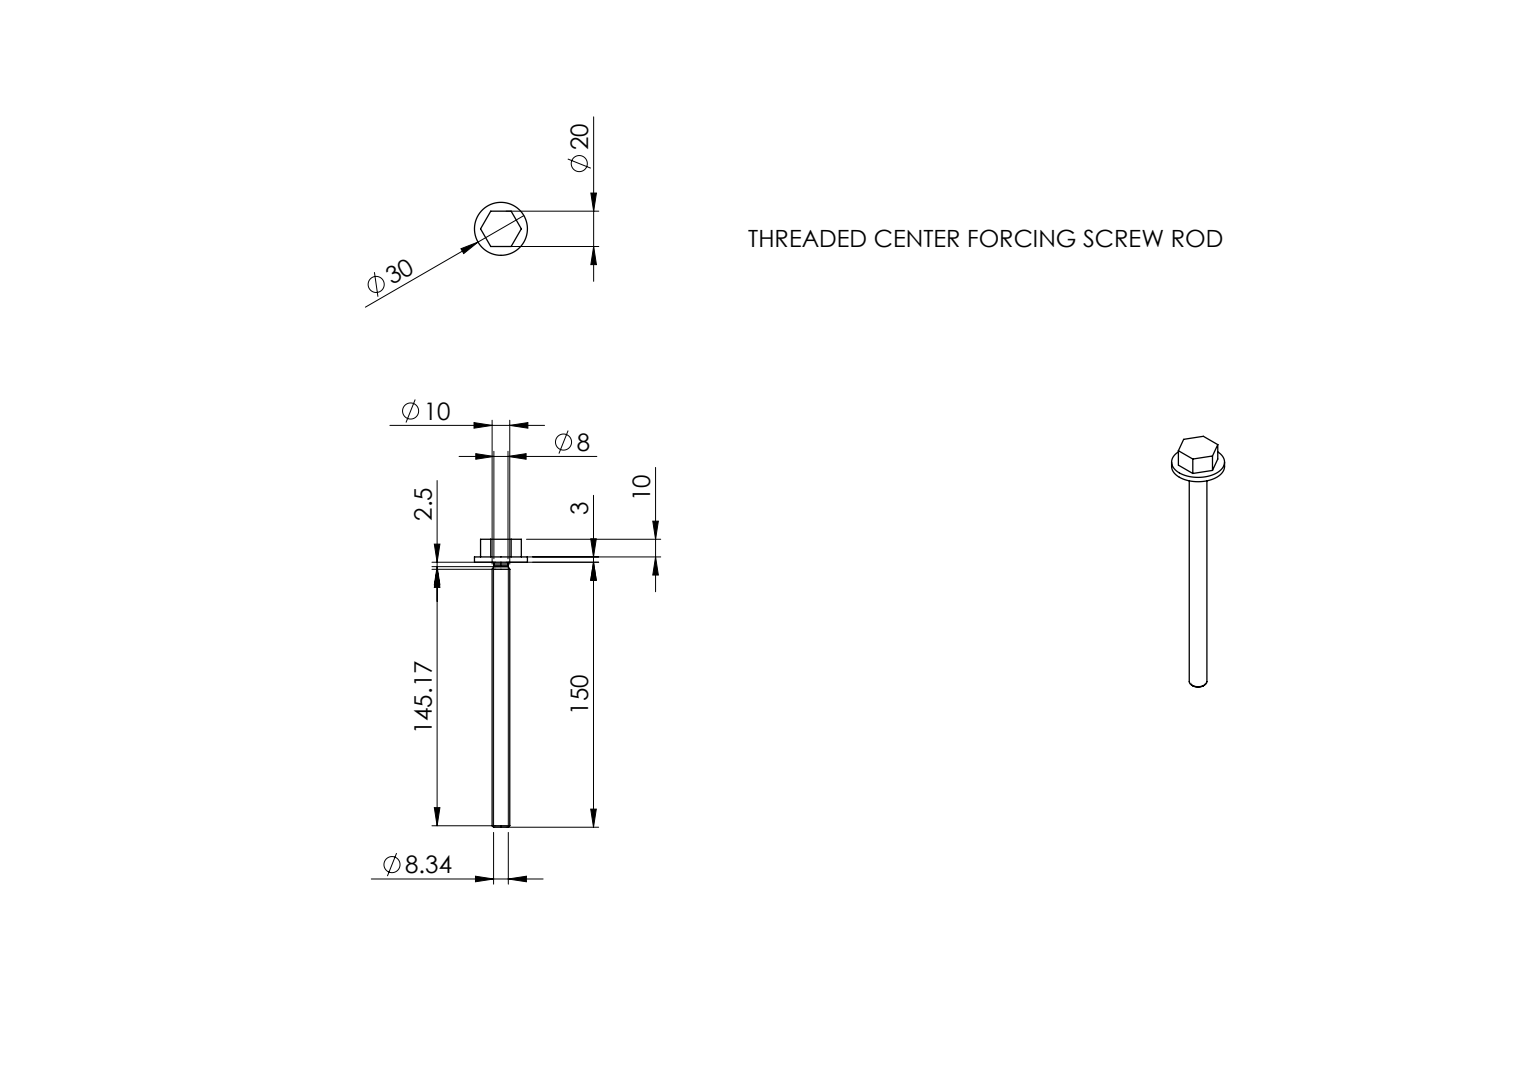
ISO-10303-21;
HEADER;
FILE_DESCRIPTION (('STEP AP214'),
    '1' );
FILE_NAME ('Threaded Center Forcing Screw Rod.step',
    '2026-10-22T13:24:12',
    ( '' ),
    ( '' ),
    'SwSTEP 2.0',
    'SolidWorks 2026',
    '' );
FILE_SCHEMA (( 'AUTOMOTIVE_DESIGN' ));
ENDSEC;

DATA;
#2=CARTESIAN_POINT ( 'NONE',  ( 0.000000000000000000, -150.0000000000000000, 0.000000000000000000 ) ) ;
#4=EDGE_CURVE ( 'NONE', #2839, #391, #2268, .T. ) ;
#5=LINE ( 'NONE', #437, #2768 ) ;
#11=AXIS2_PLACEMENT_3D ( 'NONE', #480, #2053, #1136 ) ;
#12=CARTESIAN_POINT ( 'NONE',  ( 5.510910596163087583E-16, -0.9999999999999997780, -3.999999999999999112 ) ) ;
#14=DIRECTION ( 'NONE',  ( -1.000000000000000000, 0.000000000000000000, 1.502314598737159524E-16 ) ) ;
#17=DIRECTION ( 'NONE',  ( -1.000000000000000000, 0.000000000000000000, 3.004629197474320528E-16 ) ) ;
#18=DIRECTION ( 'NONE',  ( -0.000000000000000000, -1.000000000000000000, -0.000000000000000000 ) ) ;
#24=DIRECTION ( 'NONE',  ( 0.000000000000000000, 0.7071067811865452413, 0.7071067811865497932 ) ) ;
#27=CARTESIAN_POINT ( 'NONE',  ( -5.773502691896258199, 13.00000000000000178, -9.999999999999998224 ) ) ;
#28=EDGE_CURVE ( 'NONE', #2653, #1371, #1839, .T. ) ;
#36=EDGE_CURVE ( 'NONE', #1503, #53, #2280, .T. ) ;
#39=DIRECTION ( 'NONE',  ( -1.000000000000000000, 0.000000000000000000, 0.000000000000000000 ) ) ;
#45=FACE_OUTER_BOUND ( 'NONE', #672, .T. ) ;
#46=AXIS2_PLACEMENT_3D ( 'NONE', #1452, #789, #2135 ) ;
#51=AXIS2_PLACEMENT_3D ( 'NONE', #933, #1833, #2774 ) ;
#53=VERTEX_POINT ( 'NONE', #12 ) ;
#56=CARTESIAN_POINT ( 'NONE',  ( 0.000000000000000000, -1.000000000000000000, 0.000000000000000000 ) ) ;
#71=CIRCLE ( 'NONE', #1705, 4.999999999999998224 ) ;
#74=ORIENTED_EDGE ( 'NONE', *, *, #1121, .T. ) ;
#81=VERTEX_POINT ( 'NONE', #86 ) ;
#85=ORIENTED_EDGE ( 'NONE', *, *, #1055, .F. ) ;
#86=CARTESIAN_POINT ( 'NONE',  ( 0.000000000000000000, -149.1719999999999970, 5.000000000000000000 ) ) ;
#88=ORIENTED_EDGE ( 'NONE', *, *, #2477, .T. ) ;
#90=DIRECTION ( 'NONE',  ( 0.8660254037844383745, 0.000000000000000000, -0.5000000000000004441 ) ) ;
#95=PLANE ( 'NONE',  #2598 ) ;
#96=EDGE_LOOP ( 'NONE', ( #402, #361, #2058, #215 ) ) ;
#107=VECTOR ( 'NONE', #1157, 1000.000000000000000 ) ;
#122=LINE ( 'NONE', #1519, #2601 ) ;
#126=DIRECTION ( 'NONE',  ( -0.8660254037844390407, 0.000000000000000000, -0.4999999999999993339 ) ) ;
#136=DIRECTION ( 'NONE',  ( 0.000000000000000000, 0.000000000000000000, 1.000000000000000000 ) ) ;
#137=DIRECTION ( 'NONE',  ( 0.000000000000000000, 0.000000000000000000, 1.000000000000000000 ) ) ;
#141=AXIS2_PLACEMENT_3D ( 'NONE', #801, #2592, #136 ) ;
#142=EDGE_CURVE ( 'NONE', #1729, #1249, #2519, .T. ) ;
#145=TOROIDAL_SURFACE ( 'NONE', #1548, 4.999999999999998224, 0.9999999999999995559 ) ;
#149=ORIENTED_EDGE ( 'NONE', *, *, #1965, .T. ) ;
#153=CYLINDRICAL_SURFACE ( 'NONE', #1179, 3.999999999999998224 ) ;
#164=EDGE_CURVE ( 'NONE', #1727, #2749, #1701, .T. ) ;
#172=CYLINDRICAL_SURFACE ( 'NONE', #2274, 3.999999999999998224 ) ;
#184=ORIENTED_EDGE ( 'NONE', *, *, #1754, .T. ) ;
#207=FILL_AREA_STYLE_COLOUR ( '', #2269 ) ;
#215=ORIENTED_EDGE ( 'NONE', *, *, #2027, .T. ) ;
#217=DIRECTION ( 'NONE',  ( 0.000000000000000000, -0.000000000000000000, 1.000000000000000000 ) ) ;
#222=EDGE_LOOP ( 'NONE', ( #1224, #1858, #149, #2137 ) ) ;
#226=ORIENTED_EDGE ( 'NONE', *, *, #1897, .F. ) ;
#231=CARTESIAN_POINT ( 'NONE',  ( 0.000000000000000000, 0.000000000000000000, 0.000000000000000000 ) ) ;
#236=VECTOR ( 'NONE', #2191, 1000.000000000000000 ) ;
#240=CIRCLE ( 'NONE', #693, 5.000000000000000000 ) ;
#250=ORIENTED_EDGE ( 'NONE', *, *, #1132, .T. ) ;
#253=CARTESIAN_POINT ( 'NONE',  ( -11.54700538379251107, 13.00000000000000178, 3.469741003519073858E-15 ) ) ;
#260=LINE ( 'NONE', #2310, #780 ) ;
#262=CARTESIAN_POINT ( 'NONE',  ( 0.000000000000000000, 0.000000000000000000, -15.00000000000000178 ) ) ;
#265=CARTESIAN_POINT ( 'NONE',  ( -5.773502691896248429, 3.000000000000000000, 10.00000000000000178 ) ) ;
#268=CARTESIAN_POINT ( 'NONE',  ( 5.773502691896260863, 13.00000000000000178, 9.999999999999998224 ) ) ;
#280=ADVANCED_FACE ( 'NONE', ( #1721 ), #153, .T. ) ;
#286=DIRECTION ( 'NONE',  ( 0.000000000000000000, 0.000000000000000000, 1.000000000000000000 ) ) ;
#290=EDGE_LOOP ( 'NONE', ( #622, #1114 ) ) ;
#291=AXIS2_PLACEMENT_3D ( 'NONE', #2036, #2498, #1316 ) ;
#298=DIRECTION ( 'NONE',  ( 0.4999999999999998890, 0.000000000000000000, 0.8660254037844385966 ) ) ;
#301=DIRECTION ( 'NONE',  ( -0.000000000000000000, 1.000000000000000000, -0.000000000000000000 ) ) ;
#306=CARTESIAN_POINT ( 'NONE',  ( 0.000000000000000000, 0.000000000000000000, 0.000000000000000000 ) ) ;
#309=ADVANCED_FACE ( 'NONE', ( #2460 ), #828, .T. ) ;
#310=UNCERTAINTY_MEASURE_WITH_UNIT (LENGTH_MEASURE( 1.000000000000000082E-05 ), #2495, 'distance_accuracy_value', 'NONE');
#312=PLANE ( 'NONE',  #1216 ) ;
#329=CARTESIAN_POINT ( 'NONE',  ( 5.773502691896260863, 13.00000000000000178, 9.999999999999998224 ) ) ;
#330=EDGE_LOOP ( 'NONE', ( #811, #74, #1656, #2066 ) ) ;
#337=LINE ( 'NONE', #1932, #2374 ) ;
#338=DIRECTION ( 'NONE',  ( -0.000000000000000000, 1.000000000000000000, -0.000000000000000000 ) ) ;
#342=PRODUCT_DEFINITION ( 'UNKNOWN', '', #694, #2622 ) ;
#350=CARTESIAN_POINT ( 'NONE',  ( 0.000000000000000000, -2.500000000000000444, 0.000000000000000000 ) ) ;
#351=EDGE_LOOP ( 'NONE', ( #2396, #1986, #2575, #2754 ) ) ;
#358=EDGE_LOOP ( 'NONE', ( #85, #2337, #684, #88 ) ) ;
#360=FACE_OUTER_BOUND ( 'NONE', #424, .T. ) ;
#361=ORIENTED_EDGE ( 'NONE', *, *, #1809, .F. ) ;
#365=ORIENTED_EDGE ( 'NONE', *, *, #2096, .T. ) ;
#375=EDGE_CURVE ( 'NONE', #957, #1371, #1659, .T. ) ;
#382=ORIENTED_EDGE ( 'NONE', *, *, #2069, .F. ) ;
#391=VERTEX_POINT ( 'NONE', #1838 ) ;
#402=ORIENTED_EDGE ( 'NONE', *, *, #1276, .T. ) ;
#404=LINE ( 'NONE', #1296, #697 ) ;
#405=ADVANCED_FACE ( 'NONE', ( #1352 ), #696, .T. ) ;
#406=DIRECTION ( 'NONE',  ( 0.000000000000000000, 0.000000000000000000, 1.000000000000000000 ) ) ;
#414=( NAMED_UNIT ( * ) SI_UNIT ( $, .STERADIAN. ) SOLID_ANGLE_UNIT ( ) );
#420=LINE ( 'NONE', #253, #2911 ) ;
#421=VECTOR ( 'NONE', #2760, 1000.000000000000227 ) ;
#423=CIRCLE ( 'NONE', #2414, 4.171999999999999709 ) ;
#424=EDGE_LOOP ( 'NONE', ( #674, #785, #2678, #603 ) ) ;
#428=CARTESIAN_POINT ( 'NONE',  ( 0.000000000000000000, -2.500000000000000444, 0.000000000000000000 ) ) ;
#431=( NAMED_UNIT ( * ) SI_UNIT ( $, .STERADIAN. ) SOLID_ANGLE_UNIT ( ) );
#437=CARTESIAN_POINT ( 'NONE',  ( -5.773502691896248429, 13.00000000000000178, 10.00000000000000178 ) ) ;
#447=CARTESIAN_POINT ( 'NONE',  ( 0.000000000000000000, -2.500000000000000444, 4.133974596215572284 ) ) ;
#453=DIRECTION ( 'NONE',  ( -0.000000000000000000, 1.000000000000000000, -0.000000000000000000 ) ) ;
#457=ADVANCED_FACE ( 'NONE', ( #955 ), #1807, .T. ) ;
#459=ORIENTED_EDGE ( 'NONE', *, *, #2639, .T. ) ;
#479=EDGE_CURVE ( 'NONE', #1049, #81, #1573, .T. ) ;
#480=CARTESIAN_POINT ( 'NONE',  ( 5.773502691896257311, 13.00000000000000178, -10.00000000000000000 ) ) ;
#494=LINE ( 'NONE', #2776, #516 ) ;
#499=ORIENTED_EDGE ( 'NONE', *, *, #1348, .T. ) ;
#505=DIRECTION ( 'NONE',  ( -0.000000000000000000, 1.000000000000000000, -0.000000000000000000 ) ) ;
#507=VECTOR ( 'NONE', #1679, 1000.000000000000000 ) ;
#516=VECTOR ( 'NONE', #2323, 1000.000000000000000 ) ;
#517=DIRECTION ( 'NONE',  ( -0.000000000000000000, 1.000000000000000000, -0.000000000000000000 ) ) ;
#524=DIRECTION ( 'NONE',  ( 0.4999999999999993339, 0.000000000000000000, -0.8660254037844390407 ) ) ;
#530=ORIENTED_EDGE ( 'NONE', *, *, #2477, .F. ) ;
#537=DIRECTION ( 'NONE',  ( 0.000000000000000000, -0.000000000000000000, 1.000000000000000000 ) ) ;
#541=CARTESIAN_POINT ( 'NONE',  ( 6.123233995736766282E-16, -149.1719999999999970, -5.000000000000000000 ) ) ;
#543=DIRECTION ( 'NONE',  ( 0.000000000000000000, 1.000000000000000000, 0.000000000000000000 ) ) ;
#547=FACE_OUTER_BOUND ( 'NONE', #614, .T. ) ;
#548=FACE_OUTER_BOUND ( 'NONE', #2786, .T. ) ;
#551=ORIENTED_EDGE ( 'NONE', *, *, #1102, .F. ) ;
#555=CARTESIAN_POINT ( 'NONE',  ( 0.000000000000000000, 0.000000000000000000, 3.999999999999998224 ) ) ;
#577=APPLICATION_CONTEXT ( 'automotive_design' ) ;
#579=EDGE_CURVE ( 'NONE', #2653, #2728, #1992, .T. ) ;
#603=ORIENTED_EDGE ( 'NONE', *, *, #1774, .T. ) ;
#612=CARTESIAN_POINT ( 'NONE',  ( 0.000000000000000000, -2.500000000000000444, 0.000000000000000000 ) ) ;
#613=AXIS2_PLACEMENT_3D ( 'NONE', #2778, #2490, #1152 ) ;
#614=EDGE_LOOP ( 'NONE', ( #226, #2248, #1244, #2777 ) ) ;
#622=ORIENTED_EDGE ( 'NONE', *, *, #1348, .F. ) ;
#631=EDGE_LOOP ( 'NONE', ( #499, #763, #2072, #2015 ) ) ;
#637=ORIENTED_EDGE ( 'NONE', *, *, #2069, .T. ) ;
#639=DIRECTION ( 'NONE',  ( 0.000000000000000000, 1.000000000000000000, 0.000000000000000000 ) ) ;
#641=VECTOR ( 'NONE', #1326, 1000.000000000000000 ) ;
#643=ORIENTED_EDGE ( 'NONE', *, *, #2783, .T. ) ;
#656=ORIENTED_EDGE ( 'NONE', *, *, #1809, .T. ) ;
#670=LINE ( 'NONE', #1066, #641 ) ;
#672=EDGE_LOOP ( 'NONE', ( #2930, #1394, #2851, #2536 ) ) ;
#673=CARTESIAN_POINT ( 'NONE',  ( 0.000000000000000000, 3.000000000000000000, -15.00000000000000178 ) ) ;
#674=ORIENTED_EDGE ( 'NONE', *, *, #2651, .F. ) ;
#675=CARTESIAN_POINT ( 'NONE',  ( 5.773502691896260863, 3.000000000000000000, 9.999999999999998224 ) ) ;
#684=ORIENTED_EDGE ( 'NONE', *, *, #1451, .T. ) ;
#686=DIRECTION ( 'NONE',  ( -0.000000000000000000, 1.000000000000000000, -0.000000000000000000 ) ) ;
#693=AXIS2_PLACEMENT_3D ( 'NONE', #1251, #2832, #2860 ) ;
#694=PRODUCT_DEFINITION_FORMATION_WITH_SPECIFIED_SOURCE ( 'ANY', '', #2336, .NOT_KNOWN. ) ;
#696=PLANE ( 'NONE',  #708 ) ;
#697=VECTOR ( 'NONE', #2211, 1000.000000000000000 ) ;
#700=DIRECTION ( 'NONE',  ( 0.000000000000000000, -0.8660254037844267172, -0.5000000000000207612 ) ) ;
#701=AXIS2_PLACEMENT_3D ( 'NONE', #1280, #1697, #2617 ) ;
#705=VERTEX_POINT ( 'NONE', #1582 ) ;
#708=AXIS2_PLACEMENT_3D ( 'NONE', #1588, #2746, #1605 ) ;
#709=DIRECTION ( 'NONE',  ( 1.224646799147352468E-16, 0.000000000000000000, -1.000000000000000000 ) ) ;
#710=PLANE ( 'NONE',  #2891 ) ;
#711=PLANE ( 'NONE',  #2371 ) ;
#714=ORIENTED_EDGE ( 'NONE', *, *, #1505, .F. ) ;
#720=ORIENTED_EDGE ( 'NONE', *, *, #2117, .F. ) ;
#723=DIRECTION ( 'NONE',  ( 0.000000000000000000, 0.000000000000000000, 1.000000000000000000 ) ) ;
#734=CARTESIAN_POINT ( 'NONE',  ( 0.000000000000000000, -1.999999999999980016, 0.000000000000000000 ) ) ;
#735=CARTESIAN_POINT ( 'NONE',  ( 0.000000000000000000, 0.000000000000000000, 0.000000000000000000 ) ) ;
#737=VERTEX_POINT ( 'NONE', #1314 ) ;
#745=DIRECTION ( 'NONE',  ( -0.000000000000000000, -1.000000000000000000, -0.000000000000000000 ) ) ;
#754=CLOSED_SHELL ( 'NONE', ( #2881, #457, #2145, #2721, #1585, #2277, #1625, #2040, #2699, #1248, #2372, #1234, #1321, #2735, #2694, #1354, #2112, #1825, #280, #1540, #2775, #309, #1255, #405 ) ) ;
#756=EDGE_LOOP ( 'NONE', ( #1133, #2308, #2005, #864 ) ) ;
#759=ORIENTED_EDGE ( 'NONE', *, *, #1412, .F. ) ;
#763=ORIENTED_EDGE ( 'NONE', *, *, #2164, .T. ) ;
#766=VERTEX_POINT ( 'NONE', #675 ) ;
#771=DIRECTION ( 'NONE',  ( -0.4999999999999996114, 0.000000000000000000, 0.8660254037844388186 ) ) ;
#774=FACE_OUTER_BOUND ( 'NONE', #1288, .T. ) ;
#775=DIRECTION ( 'NONE',  ( 0.000000000000000000, 0.000000000000000000, 1.000000000000000000 ) ) ;
#776=VERTEX_POINT ( 'NONE', #2729 ) ;
#780=VECTOR ( 'NONE', #700, 1000.000000000000114 ) ;
#781=DIRECTION ( 'NONE',  ( -0.4999999999999996114, 0.000000000000000000, 0.8660254037844388186 ) ) ;
#784=VECTOR ( 'NONE', #2823, 1000.000000000000114 ) ;
#785=ORIENTED_EDGE ( 'NONE', *, *, #375, .F. ) ;
#789=DIRECTION ( 'NONE',  ( -0.000000000000000000, 1.000000000000000000, -0.000000000000000000 ) ) ;
#793=DIRECTION ( 'NONE',  ( -0.000000000000000000, 1.000000000000000000, -0.000000000000000000 ) ) ;
#801=CARTESIAN_POINT ( 'NONE',  ( 0.000000000000000000, 0.000000000000000000, 0.000000000000000000 ) ) ;
#806=CYLINDRICAL_SURFACE ( 'NONE', #1212, 15.00000000000000178 ) ;
#809=DIRECTION ( 'NONE',  ( -0.000000000000000000, 1.000000000000000000, -0.000000000000000000 ) ) ;
#811=ORIENTED_EDGE ( 'NONE', *, *, #1012, .F. ) ;
#828=CYLINDRICAL_SURFACE ( 'NONE', #2090, 5.000000000000000000 ) ;
#829=VECTOR ( 'NONE', #2691, 1000.000000000000227 ) ;
#830=FACE_OUTER_BOUND ( 'NONE', #1229, .T. ) ;
#835=DIRECTION ( 'NONE',  ( 0.000000000000000000, 0.000000000000000000, -1.000000000000000000 ) ) ;
#847=DIRECTION ( 'NONE',  ( -0.000000000000000000, 1.000000000000000000, -0.000000000000000000 ) ) ;
#864=ORIENTED_EDGE ( 'NONE', *, *, #1102, .T. ) ;
#882=AXIS2_PLACEMENT_3D ( 'NONE', #2250, #639, #217 ) ;
#885=CIRCLE ( 'NONE', #2702, 15.00000000000000178 ) ;
#894=AXIS2_PLACEMENT_3D ( 'NONE', #2, #2007, #2052 ) ;
#902=AXIS2_PLACEMENT_3D ( 'NONE', #2158, #1001, #137 ) ;
#907=LINE ( 'NONE', #1297, #2385 ) ;
#911=ORIENTED_EDGE ( 'NONE', *, *, #36, .T. ) ;
#915=VERTEX_POINT ( 'NONE', #265 ) ;
#919=DIRECTION ( 'NONE',  ( -0.8660254037844387076, 0.000000000000000000, 0.4999999999999999445 ) ) ;
#933=CARTESIAN_POINT ( 'NONE',  ( 0.000000000000000000, -1.000000000000000000, 4.999999999999998224 ) ) ;
#934=CIRCLE ( 'NONE', #141, 4.999999999999998224 ) ;
#939=CIRCLE ( 'NONE', #291, 1.000000000000000000 ) ;
#943=DIRECTION ( 'NONE',  ( -0.000000000000000000, 1.000000000000000000, -0.000000000000000000 ) ) ;
#949=CARTESIAN_POINT ( 'NONE',  ( 0.000000000000000000, -0.9999999999999997780, 3.999999999999999112 ) ) ;
#950=PLANE ( 'NONE',  #2507 ) ;
#953=VECTOR ( 'NONE', #2121, 1000.000000000000000 ) ;
#955=FACE_OUTER_BOUND ( 'NONE', #1436, .T. ) ;
#957=VERTEX_POINT ( 'NONE', #961 ) ;
#958=DIRECTION ( 'NONE',  ( -0.000000000000000000, -1.000000000000000000, -0.000000000000000000 ) ) ;
#961=CARTESIAN_POINT ( 'NONE',  ( 5.062658757011871940E-16, -2.500000000000000444, -4.133974596215572284 ) ) ;
#963=CARTESIAN_POINT ( 'NONE',  ( -11.54700538379251107, 13.00000000000000178, 3.469741003519073858E-15 ) ) ;
#976=DIRECTION ( 'NONE',  ( -0.5000000000000004441, 0.000000000000000000, -0.8660254037844383745 ) ) ;
#978=CIRCLE ( 'NONE', #46, 3.999999999999999112 ) ;
#983=DIRECTION ( 'NONE',  ( -0.4999999999999993339, 0.000000000000000000, 0.8660254037844390407 ) ) ;
#990=LINE ( 'NONE', #2821, #953 ) ;
#992=CARTESIAN_POINT ( 'NONE',  ( 0.000000000000000000, -1.999999999999980016, 3.999999999999998224 ) ) ;
#1001=DIRECTION ( 'NONE',  ( -0.000000000000000000, 1.000000000000000000, -0.000000000000000000 ) ) ;
#1002=FACE_OUTER_BOUND ( 'NONE', #358, .T. ) ;
#1005=CARTESIAN_POINT ( 'NONE',  ( 0.000000000000000000, -149.1719999999999970, 0.000000000000000000 ) ) ;
#1006=ORIENTED_EDGE ( 'NONE', *, *, #1311, .F. ) ;
#1012=EDGE_CURVE ( 'NONE', #2433, #2749, #990, .T. ) ;
#1040=CARTESIAN_POINT ( 'NONE',  ( 0.000000000000000000, 0.000000000000000000, 0.000000000000000000 ) ) ;
#1045=CARTESIAN_POINT ( 'NONE',  ( 11.54700538379251107, 13.00000000000000178, -6.939586148520149327E-15 ) ) ;
#1049=VERTEX_POINT ( 'NONE', #1350 ) ;
#1055=EDGE_CURVE ( 'NONE', #1249, #1871, #1541, .T. ) ;
#1060=EDGE_LOOP ( 'NONE', ( #2209, #1680, #1329, #656 ) ) ;
#1065=EDGE_CURVE ( 'NONE', #1905, #776, #420, .T. ) ;
#1066=CARTESIAN_POINT ( 'NONE',  ( 6.123233995736766282E-16, -149.1719999999999970, -5.000000000000000000 ) ) ;
#1069=CONICAL_SURFACE ( 'NONE', #1688, 5.000000000000000000, 0.7853981633974514986 ) ;
#1070=DIRECTION ( 'NONE',  ( -0.000000000000000000, -1.000000000000000000, -0.000000000000000000 ) ) ;
#1078=CARTESIAN_POINT ( 'NONE',  ( 0.000000000000000000, -149.1719999999999970, 0.000000000000000000 ) ) ;
#1088=CIRCLE ( 'NONE', #2620, 5.000000000000000000 ) ;
#1090=SURFACE_STYLE_USAGE ( .BOTH. , #2467 ) ;
#1094=DIRECTION ( 'NONE',  ( -0.000000000000000000, 1.000000000000000000, -0.000000000000000000 ) ) ;
#1102=EDGE_CURVE ( 'NONE', #2075, #766, #907, .T. ) ;
#1108=PLANE ( 'NONE',  #1552 ) ;
#1109=DIRECTION ( 'NONE',  ( -0.000000000000000000, -1.000000000000000000, -0.000000000000000000 ) ) ;
#1113=DIRECTION ( 'NONE',  ( -0.000000000000000000, 1.000000000000000000, -0.000000000000000000 ) ) ;
#1114=ORIENTED_EDGE ( 'NONE', *, *, #1749, .F. ) ;
#1115=CONICAL_SURFACE ( 'NONE', #1495, 4.133974596215571395, 0.5235987755983229075 ) ;
#1116=DIRECTION ( 'NONE',  ( -0.000000000000000000, 1.000000000000000000, -0.000000000000000000 ) ) ;
#1118=VECTOR ( 'NONE', #781, 1000.000000000000114 ) ;
#1121=EDGE_CURVE ( 'NONE', #2433, #81, #1088, .T. ) ;
#1124=CIRCLE ( 'NONE', #2810, 5.000000000000000000 ) ;
#1126=CARTESIAN_POINT ( 'NONE',  ( 0.000000000000000000, -149.1719999999999970, 5.000000000000000000 ) ) ;
#1129=LINE ( 'NONE', #2046, #2025 ) ;
#1132=EDGE_CURVE ( 'NONE', #705, #1494, #71, .T. ) ;
#1133=ORIENTED_EDGE ( 'NONE', *, *, #2872, .T. ) ;
#1136=DIRECTION ( 'NONE',  ( 1.000000000000000000, 0.000000000000000000, -1.502314598737159524E-16 ) ) ;
#1137=PLANE ( 'NONE',  #11 ) ;
#1138=EDGE_CURVE ( 'NONE', #776, #915, #5, .T. ) ;
#1152=DIRECTION ( 'NONE',  ( 0.000000000000000000, 0.000000000000000000, 1.000000000000000000 ) ) ;
#1156=CARTESIAN_POINT ( 'NONE',  ( 0.000000000000000000, -1.999999999999980016, 4.999999999999998224 ) ) ;
#1157=DIRECTION ( 'NONE',  ( -0.000000000000000000, -1.000000000000000000, -0.000000000000000000 ) ) ;
#1160=VECTOR ( 'NONE', #745, 1000.000000000000000 ) ;
#1170=( GEOMETRIC_REPRESENTATION_CONTEXT ( 3 ) GLOBAL_UNCERTAINTY_ASSIGNED_CONTEXT ( ( #1831 ) ) GLOBAL_UNIT_ASSIGNED_CONTEXT ( ( #1477, #2599, #2403 ) ) REPRESENTATION_CONTEXT ( 'NONE', 'WORKASPACE' ) );
#1173=TOROIDAL_SURFACE ( 'NONE', #2177, 4.999999999999998224, 0.9999999999999995559 ) ;
#1176=ADVANCED_BREP_SHAPE_REPRESENTATION ( '', ( #1577, #2652 ), #2217 ) ;
#1177=ORIENTED_EDGE ( 'NONE', *, *, #2449, .F. ) ;
#1179=AXIS2_PLACEMENT_3D ( 'NONE', #1498, #847, #2190 ) ;
#1182=DIRECTION ( 'NONE',  ( 0.000000000000000000, 1.000000000000000000, 0.000000000000000000 ) ) ;
#1192=DIRECTION ( 'NONE',  ( 0.000000000000000000, 0.000000000000000000, 1.000000000000000000 ) ) ;
#1197=DIRECTION ( 'NONE',  ( 1.000000000000000000, 0.000000000000000000, 1.224646799147353207E-16 ) ) ;
#1199=LINE ( 'NONE', #268, #1313 ) ;
#1207=ORIENTED_EDGE ( 'NONE', *, *, #1276, .F. ) ;
#1209=UNCERTAINTY_MEASURE_WITH_UNIT (LENGTH_MEASURE( 1.000000000000000082E-05 ), #1985, 'distance_accuracy_value', 'NONE');
#1212=AXIS2_PLACEMENT_3D ( 'NONE', #2643, #1709, #2630 ) ;
#1216=AXIS2_PLACEMENT_3D ( 'NONE', #963, #90, #976 ) ;
#1222=MECHANICAL_DESIGN_GEOMETRIC_PRESENTATION_REPRESENTATION('',(#2563),#1170);
#1224=ORIENTED_EDGE ( 'NONE', *, *, #2639, .F. ) ;
#1226=AXIS2_PLACEMENT_3D ( 'NONE', #1911, #543, #2398 ) ;
#1229=EDGE_LOOP ( 'NONE', ( #720, #2771, #2825, #2871 ) ) ;
#1233=ORIENTED_EDGE ( 'NONE', *, *, #28, .T. ) ;
#1234=ADVANCED_FACE ( 'NONE', ( #2307 ), #2083, .F. ) ;
#1235=VECTOR ( 'NONE', #1109, 1000.000000000000000 ) ;
#1238=DIRECTION ( 'NONE',  ( -0.000000000000000000, 1.000000000000000000, -0.000000000000000000 ) ) ;
#1244=ORIENTED_EDGE ( 'NONE', *, *, #1840, .T. ) ;
#1247=LINE ( 'NONE', #555, #2262 ) ;
#1248=ADVANCED_FACE ( 'NONE', ( #2533, #2743 ), #711, .F. ) ;
#1249=VERTEX_POINT ( 'NONE', #1834 ) ;
#1251=CARTESIAN_POINT ( 'NONE',  ( 0.000000000000000000, -149.1719999999999970, 0.000000000000000000 ) ) ;
#1255=ADVANCED_FACE ( 'NONE', ( #45 ), #1463, .T. ) ;
#1260=STYLED_ITEM ( 'NONE', ( #1770 ), #1176 ) ;
#1261=CARTESIAN_POINT ( 'NONE',  ( 5.773502691896260863, 13.00000000000000178, 9.999999999999998224 ) ) ;
#1265=DIRECTION ( 'NONE',  ( 0.000000000000000000, 0.000000000000000000, 1.000000000000000000 ) ) ;
#1271=CIRCLE ( 'NONE', #1370, 15.00000000000000178 ) ;
#1276=EDGE_CURVE ( 'NONE', #1425, #737, #494, .T. ) ;
#1279=EDGE_LOOP ( 'NONE', ( #530, #2658 ) ) ;
#1280=CARTESIAN_POINT ( 'NONE',  ( 0.000000000000000000, -1.999999999999980016, 0.000000000000000000 ) ) ;
#1281=DIRECTION ( 'NONE',  ( 0.5000000000000004441, 0.000000000000000000, 0.8660254037844383745 ) ) ;
#1286=EDGE_CURVE ( 'NONE', #2075, #2839, #1199, .T. ) ;
#1288=EDGE_LOOP ( 'NONE', ( #759, #2631, #1233, #2088 ) ) ;
#1296=CARTESIAN_POINT ( 'NONE',  ( 0.000000000000000000, 3.000000000000000000, -15.00000000000000178 ) ) ;
#1297=CARTESIAN_POINT ( 'NONE',  ( 5.773502691896260863, 13.00000000000000178, 9.999999999999998224 ) ) ;
#1298=EDGE_LOOP ( 'NONE', ( #2796, #1177 ) ) ;
#1304=FACE_OUTER_BOUND ( 'NONE', #1611, .T. ) ;
#1307=AXIS2_PLACEMENT_3D ( 'NONE', #350, #1726, #835 ) ;
#1309=DIRECTION ( 'NONE',  ( 1.000000000000000000, 0.000000000000000000, 0.000000000000000000 ) ) ;
#1311=EDGE_CURVE ( 'NONE', #391, #1425, #1853, .T. ) ;
#1313=VECTOR ( 'NONE', #524, 1000.000000000000000 ) ;
#1314=CARTESIAN_POINT ( 'NONE',  ( -5.773502691896258199, 3.000000000000000000, -9.999999999999998224 ) ) ;
#1316=DIRECTION ( 'NONE',  ( 1.224646799147352468E-16, 0.000000000000000000, -1.000000000000000000 ) ) ;
#1321=ADVANCED_FACE ( 'NONE', ( #2354 ), #1137, .F. ) ;
#1326=DIRECTION ( 'NONE',  ( 8.659560562354961208E-17, 0.7071067811865452413, -0.7071067811865497932 ) ) ;
#1329=ORIENTED_EDGE ( 'NONE', *, *, #2351, .F. ) ;
#1340=LINE ( 'NONE', #1734, #236 ) ;
#1348=EDGE_CURVE ( 'NONE', #1049, #2555, #2607, .T. ) ;
#1350=CARTESIAN_POINT ( 'NONE',  ( 0.000000000000000000, -150.0000000000000000, 4.171999999999999709 ) ) ;
#1352=FACE_OUTER_BOUND ( 'NONE', #290, .T. ) ;
#1353=SHAPE_DEFINITION_REPRESENTATION ( #1870, #1689 ) ;
#1354=ADVANCED_FACE ( 'NONE', ( #2487 ), #1108, .F. ) ;
#1356=AXIS2_PLACEMENT_3D ( 'NONE', #1821, #453, #286 ) ;
#1357=ORIENTED_EDGE ( 'NONE', *, *, #1012, .T. ) ;
#1359=CARTESIAN_POINT ( 'NONE',  ( 0.000000000000000000, -150.0000000000000000, 0.000000000000000000 ) ) ;
#1361=ORIENTED_EDGE ( 'NONE', *, *, #1897, .T. ) ;
#1362=CIRCLE ( 'NONE', #1460, 3.999999999999998224 ) ;
#1366=CARTESIAN_POINT ( 'NONE',  ( 5.773502691896257311, 3.000000000000000000, -10.00000000000000000 ) ) ;
#1370=AXIS2_PLACEMENT_3D ( 'NONE', #306, #1845, #1192 ) ;
#1371=VERTEX_POINT ( 'NONE', #447 ) ;
#1372=DIRECTION ( 'NONE',  ( -0.000000000000000000, 1.000000000000000000, -0.000000000000000000 ) ) ;
#1392=DIRECTION ( 'NONE',  ( 0.000000000000000000, 0.000000000000000000, 1.000000000000000000 ) ) ;
#1394=ORIENTED_EDGE ( 'NONE', *, *, #1749, .T. ) ;
#1398=LINE ( 'NONE', #1864, #2504 ) ;
#1409=CIRCLE ( 'NONE', #2885, 15.00000000000000178 ) ;
#1412=EDGE_CURVE ( 'NONE', #2728, #957, #939, .T. ) ;
#1422=AXIS2_PLACEMENT_3D ( 'NONE', #2726, #1070, #2483 ) ;
#1425=VERTEX_POINT ( 'NONE', #1366 ) ;
#1426=CARTESIAN_POINT ( 'NONE',  ( -5.773502691896258199, 13.00000000000000178, -9.999999999999998224 ) ) ;
#1436=EDGE_LOOP ( 'NONE', ( #643, #1357, #2693, #2857 ) ) ;
#1437=DIRECTION ( 'NONE',  ( 0.000000000000000000, 0.000000000000000000, 1.000000000000000000 ) ) ;
#1451=EDGE_CURVE ( 'NONE', #1729, #1842, #404, .T. ) ;
#1452=CARTESIAN_POINT ( 'NONE',  ( 0.000000000000000000, -0.9999999999999997780, 0.000000000000000000 ) ) ;
#1455=CARTESIAN_POINT ( 'NONE',  ( 0.000000000000000000, -1.999999999999980016, 0.000000000000000000 ) ) ;
#1457=ORIENTED_EDGE ( 'NONE', *, *, #28, .F. ) ;
#1460=AXIS2_PLACEMENT_3D ( 'NONE', #734, #338, #2063 ) ;
#1463=CONICAL_SURFACE ( 'NONE', #2174, 5.000000000000000000, 0.7853981633974514986 ) ;
#1477=( LENGTH_UNIT ( ) NAMED_UNIT ( * ) SI_UNIT ( .MILLI., .METRE. ) );
#1481=ORIENTED_EDGE ( 'NONE', *, *, #1138, .T. ) ;
#1487=DIRECTION ( 'NONE',  ( 1.000000000000000000, 0.000000000000000000, -3.004629197474320528E-16 ) ) ;
#1494=VERTEX_POINT ( 'NONE', #1644 ) ;
#1495=AXIS2_PLACEMENT_3D ( 'NONE', #612, #2708, #2900 ) ;
#1498=CARTESIAN_POINT ( 'NONE',  ( 0.000000000000000000, 0.000000000000000000, 0.000000000000000000 ) ) ;
#1500=CONICAL_SURFACE ( 'NONE', #1307, 4.133974596215571395, 0.5235987755983229075 ) ;
#1503=VERTEX_POINT ( 'NONE', #949 ) ;
#1505=EDGE_CURVE ( 'NONE', #1494, #53, #2224, .T. ) ;
#1513=DIRECTION ( 'NONE',  ( -0.000000000000000000, 1.000000000000000000, -0.000000000000000000 ) ) ;
#1515=PRODUCT_CONTEXT ( 'NONE', #577, 'mechanical' ) ;
#1519=CARTESIAN_POINT ( 'NONE',  ( 5.773502691896260863, 3.000000000000000000, 9.999999999999998224 ) ) ;
#1540=ADVANCED_FACE ( 'NONE', ( #774 ), #2465, .F. ) ;
#1541=LINE ( 'NONE', #2455, #1235 ) ;
#1545=DIRECTION ( 'NONE',  ( 0.000000000000000000, 0.000000000000000000, 1.000000000000000000 ) ) ;
#1548=AXIS2_PLACEMENT_3D ( 'NONE', #1455, #2367, #723 ) ;
#1552=AXIS2_PLACEMENT_3D ( 'NONE', #2684, #2714, #17 ) ;
#1560=EDGE_CURVE ( 'NONE', #81, #1727, #337, .T. ) ;
#1570=ORIENTED_EDGE ( 'NONE', *, *, #1967, .T. ) ;
#1573=LINE ( 'NONE', #1126, #2856 ) ;
#1577=MANIFOLD_SOLID_BREP ( 'M10 Machine Threads Stud1', #754 ) ;
#1580=( NAMED_UNIT ( * ) PLANE_ANGLE_UNIT ( ) SI_UNIT ( $, .RADIAN. ) );
#1582=CARTESIAN_POINT ( 'NONE',  ( 0.000000000000000000, -2.168404344971008868E-16, 4.999999999999998224 ) ) ;
#1585=ADVANCED_FACE ( 'NONE', ( #2859 ), #172, .T. ) ;
#1588=CARTESIAN_POINT ( 'NONE',  ( 4.171999999999999709, -150.0000000000000000, 0.000000000000000000 ) ) ;
#1590=VECTOR ( 'NONE', #1487, 1000.000000000000000 ) ;
#1593=CARTESIAN_POINT ( 'NONE',  ( -11.54700538379251107, 13.00000000000000178, 3.469741003519073858E-15 ) ) ;
#1601=ORIENTED_EDGE ( 'NONE', *, *, #1965, .F. ) ;
#1604=ORIENTED_EDGE ( 'NONE', *, *, #2732, .F. ) ;
#1605=DIRECTION ( 'NONE',  ( 0.000000000000000000, -0.000000000000000000, -1.000000000000000000 ) ) ;
#1611=EDGE_LOOP ( 'NONE', ( #1682, #1948, #184, #2392, #1977, #637 ) ) ;
#1614=CARTESIAN_POINT ( 'NONE',  ( -5.773502691896258199, 13.00000000000000178, -9.999999999999998224 ) ) ;
#1616=DIRECTION ( 'NONE',  ( 0.000000000000000000, 0.000000000000000000, 1.000000000000000000 ) ) ;
#1624=DIRECTION ( 'NONE',  ( 0.000000000000000000, 0.000000000000000000, 1.000000000000000000 ) ) ;
#1625=ADVANCED_FACE ( 'NONE', ( #547 ), #2366, .T. ) ;
#1633=ORIENTED_EDGE ( 'NONE', *, *, #1065, .F. ) ;
#1641=EDGE_LOOP ( 'NONE', ( #714, #2345, #1793, #911 ) ) ;
#1644=CARTESIAN_POINT ( 'NONE',  ( 6.123233995736764310E-16, -2.168404344971008868E-16, -4.999999999999998224 ) ) ;
#1646=CARTESIAN_POINT ( 'NONE',  ( 11.54700538379251107, 13.00000000000000178, -6.939586148520149327E-15 ) ) ;
#1656=ORIENTED_EDGE ( 'NONE', *, *, #1560, .T. ) ;
#1659=CIRCLE ( 'NONE', #613, 4.133974596215571395 ) ;
#1661=LINE ( 'NONE', #2589, #784 ) ;
#1664=ORIENTED_EDGE ( 'NONE', *, *, #2845, .F. ) ;
#1674=FACE_BOUND ( 'NONE', #2662, .T. ) ;
#1679=DIRECTION ( 'NONE',  ( -0.000000000000000000, -1.000000000000000000, -0.000000000000000000 ) ) ;
#1680=ORIENTED_EDGE ( 'NONE', *, *, #1914, .F. ) ;
#1682=ORIENTED_EDGE ( 'NONE', *, *, #1286, .T. ) ;
#1688=AXIS2_PLACEMENT_3D ( 'NONE', #1005, #1907, #775 ) ;
#1689=SHAPE_REPRESENTATION ( 'Threaded Center Forcing Screw Rod', ( #2652 ), #2217 ) ;
#1697=DIRECTION ( 'NONE',  ( -0.000000000000000000, 1.000000000000000000, -0.000000000000000000 ) ) ;
#1701=CIRCLE ( 'NONE', #902, 5.000000000000000000 ) ;
#1705=AXIS2_PLACEMENT_3D ( 'NONE', #2913, #2500, #406 ) ;
#1709=DIRECTION ( 'NONE',  ( -0.000000000000000000, -1.000000000000000000, -0.000000000000000000 ) ) ;
#1721=FACE_OUTER_BOUND ( 'NONE', #222, .T. ) ;
#1726=DIRECTION ( 'NONE',  ( 0.000000000000000000, -1.000000000000000000, 0.000000000000000000 ) ) ;
#1727=VERTEX_POINT ( 'NONE', #2924 ) ;
#1729=VERTEX_POINT ( 'NONE', #673 ) ;
#1734=CARTESIAN_POINT ( 'NONE',  ( -5.773502691896248429, 3.000000000000000000, 10.00000000000000178 ) ) ;
#1735=AXIS2_PLACEMENT_3D ( 'NONE', #1646, #919, #298 ) ;
#1740=DIRECTION ( 'NONE',  ( 0.000000000000000000, 0.000000000000000000, 1.000000000000000000 ) ) ;
#1745=DIRECTION ( 'NONE',  ( -0.000000000000000000, -1.000000000000000000, -0.000000000000000000 ) ) ;
#1749=EDGE_CURVE ( 'NONE', #2555, #1049, #423, .T. ) ;
#1754=EDGE_CURVE ( 'NONE', #2644, #1806, #2665, .T. ) ;
#1767=CARTESIAN_POINT ( 'NONE',  ( 11.54700538379251107, 13.00000000000000178, -6.939586148520149327E-15 ) ) ;
#1768=ORIENTED_EDGE ( 'NONE', *, *, #2845, .T. ) ;
#1770=PRESENTATION_STYLE_ASSIGNMENT (( #1090 ) ) ;
#1774=EDGE_CURVE ( 'NONE', #2749, #1727, #1124, .T. ) ;
#1793=ORIENTED_EDGE ( 'NONE', *, *, #2732, .T. ) ;
#1798=CARTESIAN_POINT ( 'NONE',  ( 5.773502691896257311, 13.00000000000000178, -10.00000000000000000 ) ) ;
#1806=VERTEX_POINT ( 'NONE', #27 ) ;
#1807=CYLINDRICAL_SURFACE ( 'NONE', #2905, 5.000000000000000000 ) ;
#1809=EDGE_CURVE ( 'NONE', #1806, #737, #2287, .T. ) ;
#1811=DIRECTION ( 'NONE',  ( 0.000000000000000000, 0.000000000000000000, 1.000000000000000000 ) ) ;
#1812=SHAPE_REPRESENTATION_RELATIONSHIP ( 'NONE' , 'NONE' ,  #1689, #1176 ) ;
#1817=CARTESIAN_POINT ( 'NONE',  ( 0.000000000000000000, -149.1719999999999970, 0.000000000000000000 ) ) ;
#1821=CARTESIAN_POINT ( 'NONE',  ( 0.000000000000000000, -1.000000000000000000, 0.000000000000000000 ) ) ;
#1825=ADVANCED_FACE ( 'NONE', ( #2074 ), #1173, .F. ) ;
#1829=CIRCLE ( 'NONE', #51, 1.000000000000000000 ) ;
#1831=UNCERTAINTY_MEASURE_WITH_UNIT (LENGTH_MEASURE( 1.000000000000000082E-05 ), #1477, 'distance_accuracy_value', 'NONE');
#1833=DIRECTION ( 'NONE',  ( -1.000000000000000000, 0.000000000000000000, 0.000000000000000000 ) ) ;
#1834=CARTESIAN_POINT ( 'NONE',  ( 1.836970198721029983E-15, 3.000000000000000000, 15.00000000000000178 ) ) ;
#1838=CARTESIAN_POINT ( 'NONE',  ( 11.54700538379251107, 3.000000000000000000, -6.939586148520149327E-15 ) ) ;
#1839=CIRCLE ( 'NONE', #2329, 1.000000000000000000 ) ;
#1840=EDGE_CURVE ( 'NONE', #1871, #1842, #1271, .T. ) ;
#1842=VERTEX_POINT ( 'NONE', #262 ) ;
#1843=DIRECTION ( 'NONE',  ( 0.000000000000000000, 0.000000000000000000, 1.000000000000000000 ) ) ;
#1845=DIRECTION ( 'NONE',  ( 0.000000000000000000, 1.000000000000000000, 0.000000000000000000 ) ) ;
#1852=CARTESIAN_POINT ( 'NONE',  ( 0.000000000000000000, 3.000000000000000000, 0.000000000000000000 ) ) ;
#1853=LINE ( 'NONE', #2518, #421 ) ;
#1858=ORIENTED_EDGE ( 'NONE', *, *, #2722, .T. ) ;
#1860=CARTESIAN_POINT ( 'NONE',  ( 1.836970198721029983E-15, 0.000000000000000000, 15.00000000000000178 ) ) ;
#1864=CARTESIAN_POINT ( 'NONE',  ( 4.898587196589410857E-16, 0.000000000000000000, -3.999999999999998224 ) ) ;
#1865=DIRECTION ( 'NONE',  ( -0.000000000000000000, 1.000000000000000000, -0.000000000000000000 ) ) ;
#1870=PRODUCT_DEFINITION_SHAPE ( 'NONE', 'NONE',  #342 ) ;
#1871=VERTEX_POINT ( 'NONE', #1860 ) ;
#1873=LINE ( 'NONE', #2803, #1160 ) ;
#1874=TOROIDAL_SURFACE ( 'NONE', #1356, 4.999999999999998224, 0.9999999999999995559 ) ;
#1879=FACE_OUTER_BOUND ( 'NONE', #1898, .T. ) ;
#1892=EDGE_LOOP ( 'NONE', ( #2849, #459, #2162, #1601 ) ) ;
#1897=EDGE_CURVE ( 'NONE', #1249, #1729, #1409, .T. ) ;
#1898=EDGE_LOOP ( 'NONE', ( #1909, #1361 ) ) ;
#1901=CARTESIAN_POINT ( 'NONE',  ( -5.773502691896258199, 13.00000000000000178, -9.999999999999998224 ) ) ;
#1905=VERTEX_POINT ( 'NONE', #1593 ) ;
#1907=DIRECTION ( 'NONE',  ( -0.000000000000000000, 1.000000000000000000, -0.000000000000000000 ) ) ;
#1909=ORIENTED_EDGE ( 'NONE', *, *, #142, .T. ) ;
#1911=CARTESIAN_POINT ( 'NONE',  ( 0.000000000000000000, 3.000000000000000000, 0.000000000000000000 ) ) ;
#1912=LINE ( 'NONE', #2837, #1590 ) ;
#1914=EDGE_CURVE ( 'NONE', #1905, #2512, #1873, .T. ) ;
#1918=CIRCLE ( 'NONE', #2168, 4.133974596215571395 ) ;
#1928=EDGE_CURVE ( 'NONE', #737, #2512, #1129, .T. ) ;
#1930=CARTESIAN_POINT ( 'NONE',  ( 5.773502691896257311, 13.00000000000000178, -10.00000000000000000 ) ) ;
#1932=CARTESIAN_POINT ( 'NONE',  ( 0.000000000000000000, 0.000000000000000000, 5.000000000000000000 ) ) ;
#1944=DIRECTION ( 'NONE',  ( 0.000000000000000000, 1.000000000000000000, 0.000000000000000000 ) ) ;
#1948=ORIENTED_EDGE ( 'NONE', *, *, #2200, .T. ) ;
#1950=LINE ( 'NONE', #2874, #2805 ) ;
#1958=DIRECTION ( 'NONE',  ( 0.000000000000000000, 0.000000000000000000, 1.000000000000000000 ) ) ;
#1965=EDGE_CURVE ( 'NONE', #2653, #1503, #1247, .T. ) ;
#1967=EDGE_CURVE ( 'NONE', #53, #1503, #978, .T. ) ;
#1977=ORIENTED_EDGE ( 'NONE', *, *, #1065, .T. ) ;
#1982=ORIENTED_EDGE ( 'NONE', *, *, #375, .T. ) ;
#1985=( LENGTH_UNIT ( ) NAMED_UNIT ( * ) SI_UNIT ( .MILLI., .METRE. ) );
#1986=ORIENTED_EDGE ( 'NONE', *, *, #2027, .F. ) ;
#1992=CIRCLE ( 'NONE', #2764, 3.999999999999998224 ) ;
#2005=ORIENTED_EDGE ( 'NONE', *, *, #1286, .F. ) ;
#2007=DIRECTION ( 'NONE',  ( -0.000000000000000000, 1.000000000000000000, -0.000000000000000000 ) ) ;
#2015=ORIENTED_EDGE ( 'NONE', *, *, #479, .F. ) ;
#2024=DIRECTION ( 'NONE',  ( 0.000000000000000000, 0.000000000000000000, 1.000000000000000000 ) ) ;
#2025=VECTOR ( 'NONE', #771, 1000.000000000000114 ) ;
#2027=EDGE_CURVE ( 'NONE', #2644, #1425, #2818, .T. ) ;
#2031=DIRECTION ( 'NONE',  ( 0.000000000000000000, 0.000000000000000000, 1.000000000000000000 ) ) ;
#2036=CARTESIAN_POINT ( 'NONE',  ( 6.123233995736764310E-16, -1.999999999999980016, -4.999999999999998224 ) ) ;
#2039=DIRECTION ( 'NONE',  ( 0.000000000000000000, 0.000000000000000000, 1.000000000000000000 ) ) ;
#2040=ADVANCED_FACE ( 'NONE', ( #1002 ), #806, .T. ) ;
#2046=CARTESIAN_POINT ( 'NONE',  ( -5.773502691896258199, 3.000000000000000000, -9.999999999999998224 ) ) ;
#2047=SURFACE_STYLE_FILL_AREA ( #2727 ) ;
#2052=DIRECTION ( 'NONE',  ( 0.000000000000000000, 0.000000000000000000, 1.000000000000000000 ) ) ;
#2053=DIRECTION ( 'NONE',  ( 1.502314598737159524E-16, -0.000000000000000000, 1.000000000000000000 ) ) ;
#2058=ORIENTED_EDGE ( 'NONE', *, *, #1754, .F. ) ;
#2063=DIRECTION ( 'NONE',  ( 0.000000000000000000, 0.000000000000000000, 1.000000000000000000 ) ) ;
#2066=ORIENTED_EDGE ( 'NONE', *, *, #1774, .F. ) ;
#2069=EDGE_CURVE ( 'NONE', #776, #2075, #1912, .T. ) ;
#2072=ORIENTED_EDGE ( 'NONE', *, *, #2783, .F. ) ;
#2074=FACE_OUTER_BOUND ( 'NONE', #1641, .T. ) ;
#2075=VERTEX_POINT ( 'NONE', #1261 ) ;
#2080=CARTESIAN_POINT ( 'NONE',  ( 5.773502691896257311, 13.00000000000000178, -10.00000000000000000 ) ) ;
#2083=PLANE ( 'NONE',  #1735 ) ;
#2084=VECTOR ( 'NONE', #14, 1000.000000000000000 ) ;
#2088=ORIENTED_EDGE ( 'NONE', *, *, #2117, .T. ) ;
#2090=AXIS2_PLACEMENT_3D ( 'NONE', #2219, #1513, #1958 ) ;
#2096=EDGE_CURVE ( 'NONE', #915, #766, #1340, .T. ) ;
#2105=CARTESIAN_POINT ( 'NONE',  ( 0.000000000000000000, 3.000000000000000000, 0.000000000000000000 ) ) ;
#2109=FACE_OUTER_BOUND ( 'NONE', #2527, .T. ) ;
#2112=ADVANCED_FACE ( 'NONE', ( #1304 ), #2661, .T. ) ;
#2117=EDGE_CURVE ( 'NONE', #1371, #957, #1918, .T. ) ;
#2121=DIRECTION ( 'NONE',  ( -0.000000000000000000, 1.000000000000000000, -0.000000000000000000 ) ) ;
#2126=ORIENTED_EDGE ( 'NONE', *, *, #2096, .F. ) ;
#2134=VECTOR ( 'NONE', #958, 1000.000000000000000 ) ;
#2135=DIRECTION ( 'NONE',  ( 0.000000000000000000, 0.000000000000000000, 1.000000000000000000 ) ) ;
#2137=ORIENTED_EDGE ( 'NONE', *, *, #1967, .F. ) ;
#2139=FACE_OUTER_BOUND ( 'NONE', #631, .T. ) ;
#2145=ADVANCED_FACE ( 'NONE', ( #830 ), #1115, .T. ) ;
#2158=CARTESIAN_POINT ( 'NONE',  ( 0.000000000000000000, -3.999999999999900524, 0.000000000000000000 ) ) ;
#2162=ORIENTED_EDGE ( 'NONE', *, *, #36, .F. ) ;
#2164=EDGE_CURVE ( 'NONE', #2555, #2433, #670, .T. ) ;
#2168=AXIS2_PLACEMENT_3D ( 'NONE', #428, #1113, #1545 ) ;
#2174=AXIS2_PLACEMENT_3D ( 'NONE', #1817, #1865, #1616 ) ;
#2177=AXIS2_PLACEMENT_3D ( 'NONE', #56, #517, #2334 ) ;
#2190=DIRECTION ( 'NONE',  ( 0.000000000000000000, 0.000000000000000000, 1.000000000000000000 ) ) ;
#2191=DIRECTION ( 'NONE',  ( 1.000000000000000000, 0.000000000000000000, -3.004629197474320528E-16 ) ) ;
#2197=EDGE_LOOP ( 'NONE', ( #250, #2673, #1570, #1604 ) ) ;
#2200=EDGE_CURVE ( 'NONE', #2839, #2644, #2921, .T. ) ;
#2209=ORIENTED_EDGE ( 'NONE', *, *, #1928, .T. ) ;
#2211=DIRECTION ( 'NONE',  ( -0.000000000000000000, -1.000000000000000000, -0.000000000000000000 ) ) ;
#2217=( GEOMETRIC_REPRESENTATION_CONTEXT ( 3 ) GLOBAL_UNCERTAINTY_ASSIGNED_CONTEXT ( ( #310 ) ) GLOBAL_UNIT_ASSIGNED_CONTEXT ( ( #2495, #2484, #414 ) ) REPRESENTATION_CONTEXT ( 'NONE', 'WORKASPACE' ) );
#2219=CARTESIAN_POINT ( 'NONE',  ( 0.000000000000000000, 0.000000000000000000, 0.000000000000000000 ) ) ;
#2224=CIRCLE ( 'NONE', #2322, 1.000000000000000000 ) ;
#2247=EDGE_CURVE ( 'NONE', #957, #2749, #260, .T. ) ;
#2248=ORIENTED_EDGE ( 'NONE', *, *, #1055, .T. ) ;
#2250=CARTESIAN_POINT ( 'NONE',  ( 0.000000000000000000, 13.00000000000000178, 0.000000000000000000 ) ) ;
#2260=ORIENTED_EDGE ( 'NONE', *, *, #1138, .F. ) ;
#2262=VECTOR ( 'NONE', #1238, 1000.000000000000000 ) ;
#2268=LINE ( 'NONE', #2508, #2134 ) ;
#2269=COLOUR_RGB ( '',0.8941176470588234615, 0.8941176470588234615, 0.8941176470588234615 ) ;
#2274=AXIS2_PLACEMENT_3D ( 'NONE', #2646, #809, #1265 ) ;
#2277=ADVANCED_FACE ( 'NONE', ( #2299 ), #1874, .F. ) ;
#2280=CIRCLE ( 'NONE', #2418, 3.999999999999999112 ) ;
#2287=LINE ( 'NONE', #1426, #107 ) ;
#2294=CARTESIAN_POINT ( 'NONE',  ( -11.54700538379251107, 3.000000000000000000, 3.469741003519073858E-15 ) ) ;
#2298=CARTESIAN_POINT ( 'NONE',  ( 0.000000000000000000, 0.000000000000000000, 0.000000000000000000 ) ) ;
#2299=FACE_OUTER_BOUND ( 'NONE', #2197, .T. ) ;
#2307=FACE_OUTER_BOUND ( 'NONE', #351, .T. ) ;
#2308=ORIENTED_EDGE ( 'NONE', *, *, #4, .F. ) ;
#2310=CARTESIAN_POINT ( 'NONE',  ( 0.000000000000000000, -2.500000000000000444, -4.133974596215571395 ) ) ;
#2322=AXIS2_PLACEMENT_3D ( 'NONE', #2531, #1197, #709 ) ;
#2323=DIRECTION ( 'NONE',  ( -1.000000000000000000, 0.000000000000000000, 1.502314598737159524E-16 ) ) ;
#2329=AXIS2_PLACEMENT_3D ( 'NONE', #1156, #39, #1392 ) ;
#2332=CARTESIAN_POINT ( 'NONE',  ( 0.000000000000000000, -0.9999999999999997780, 0.000000000000000000 ) ) ;
#2334=DIRECTION ( 'NONE',  ( 0.000000000000000000, 0.000000000000000000, 1.000000000000000000 ) ) ;
#2336=PRODUCT ( 'Threaded Center Forcing Screw Rod', 'Threaded Center Forcing Screw Rod', '', ( #1515 ) ) ;
#2337=ORIENTED_EDGE ( 'NONE', *, *, #142, .F. ) ;
#2344=FACE_OUTER_BOUND ( 'NONE', #756, .T. ) ;
#2345=ORIENTED_EDGE ( 'NONE', *, *, #2449, .T. ) ;
#2351=EDGE_CURVE ( 'NONE', #1806, #1905, #2835, .T. ) ;
#2354=FACE_OUTER_BOUND ( 'NONE', #96, .T. ) ;
#2366=CYLINDRICAL_SURFACE ( 'NONE', #1422, 15.00000000000000178 ) ;
#2367=DIRECTION ( 'NONE',  ( -0.000000000000000000, 1.000000000000000000, -0.000000000000000000 ) ) ;
#2371=AXIS2_PLACEMENT_3D ( 'NONE', #735, #1182, #2809 ) ;
#2372=ADVANCED_FACE ( 'NONE', ( #2344 ), #95, .F. ) ;
#2374=VECTOR ( 'NONE', #793, 1000.000000000000000 ) ;
#2385=VECTOR ( 'NONE', #1745, 1000.000000000000000 ) ;
#2386=CARTESIAN_POINT ( 'NONE',  ( 0.000000000000000000, -1.999999999999980016, 0.000000000000000000 ) ) ;
#2392=ORIENTED_EDGE ( 'NONE', *, *, #2351, .T. ) ;
#2393=DIRECTION ( 'NONE',  ( 0.8660254037844389297, -0.000000000000000000, 0.4999999999999996114 ) ) ;
#2396=ORIENTED_EDGE ( 'NONE', *, *, #1311, .T. ) ;
#2398=DIRECTION ( 'NONE',  ( 0.000000000000000000, 0.000000000000000000, 1.000000000000000000 ) ) ;
#2403=( NAMED_UNIT ( * ) SI_UNIT ( $, .STERADIAN. ) SOLID_ANGLE_UNIT ( ) );
#2404=CARTESIAN_POINT ( 'NONE',  ( 0.000000000000000000, -3.999999999999900524, -5.000000000000000000 ) ) ;
#2409=MECHANICAL_DESIGN_GEOMETRIC_PRESENTATION_REPRESENTATION('',(#1260),#2843);
#2414=AXIS2_PLACEMENT_3D ( 'NONE', #1359, #1116, #1740 ) ;
#2418=AXIS2_PLACEMENT_3D ( 'NONE', #2332, #943, #1843 ) ;
#2421=DIRECTION ( 'NONE',  ( 0.000000000000000000, 0.000000000000000000, 1.000000000000000000 ) ) ;
#2424=APPLICATION_CONTEXT ( 'automotive_design' ) ;
#2427=CARTESIAN_POINT ( 'NONE',  ( 5.616230220889761452E-16, -150.0000000000000000, -4.171999999999999709 ) ) ;
#2433=VERTEX_POINT ( 'NONE', #541 ) ;
#2435=DIRECTION ( 'NONE',  ( 0.4999999999999993339, 0.000000000000000000, -0.8660254037844390407 ) ) ;
#2449=EDGE_CURVE ( 'NONE', #1494, #705, #934, .T. ) ;
#2455=CARTESIAN_POINT ( 'NONE',  ( 1.836970198721029983E-15, 3.000000000000000000, 15.00000000000000178 ) ) ;
#2460=FACE_OUTER_BOUND ( 'NONE', #330, .T. ) ;
#2464=ORIENTED_EDGE ( 'NONE', *, *, #1928, .F. ) ;
#2465=TOROIDAL_SURFACE ( 'NONE', #701, 4.999999999999998224, 0.9999999999999995559 ) ;
#2467=SURFACE_SIDE_STYLE ('',( #2047 ) ) ;
#2477=EDGE_CURVE ( 'NONE', #1842, #1871, #885, .T. ) ;
#2483=DIRECTION ( 'NONE',  ( 0.000000000000000000, 0.000000000000000000, -1.000000000000000000 ) ) ;
#2484=( NAMED_UNIT ( * ) PLANE_ANGLE_UNIT ( ) SI_UNIT ( $, .RADIAN. ) );
#2485=EDGE_LOOP ( 'NONE', ( #365, #551, #382, #1481 ) ) ;
#2487=FACE_OUTER_BOUND ( 'NONE', #2485, .T. ) ;
#2490=DIRECTION ( 'NONE',  ( -0.000000000000000000, 1.000000000000000000, -0.000000000000000000 ) ) ;
#2495=( LENGTH_UNIT ( ) NAMED_UNIT ( * ) SI_UNIT ( .MILLI., .METRE. ) );
#2498=DIRECTION ( 'NONE',  ( 1.000000000000000000, 0.000000000000000000, 1.224646799147353207E-16 ) ) ;
#2500=DIRECTION ( 'NONE',  ( 0.000000000000000000, -1.000000000000000000, 0.000000000000000000 ) ) ;
#2504=VECTOR ( 'NONE', #505, 1000.000000000000000 ) ;
#2507=AXIS2_PLACEMENT_3D ( 'NONE', #1852, #2577, #537 ) ;
#2508=CARTESIAN_POINT ( 'NONE',  ( 11.54700538379251107, 13.00000000000000178, -6.939586148520149327E-15 ) ) ;
#2512=VERTEX_POINT ( 'NONE', #2294 ) ;
#2518=CARTESIAN_POINT ( 'NONE',  ( 11.54700538379251107, 3.000000000000000000, -6.939586148520149327E-15 ) ) ;
#2519=CIRCLE ( 'NONE', #1226, 15.00000000000000178 ) ;
#2521=ORIENTED_EDGE ( 'NONE', *, *, #2872, .F. ) ;
#2527=EDGE_LOOP ( 'NONE', ( #1768, #2260, #1633, #2725 ) ) ;
#2531=CARTESIAN_POINT ( 'NONE',  ( 6.123233995736764310E-16, -1.000000000000000000, -4.999999999999998224 ) ) ;
#2533=FACE_BOUND ( 'NONE', #1298, .T. ) ;
#2536=ORIENTED_EDGE ( 'NONE', *, *, #1121, .F. ) ;
#2555=VERTEX_POINT ( 'NONE', #2427 ) ;
#2559=CARTESIAN_POINT ( 'NONE',  ( 4.898587196589410857E-16, -1.999999999999980016, -3.999999999999998224 ) ) ;
#2563=STYLED_ITEM('',(#2970),#1577);
#2575=ORIENTED_EDGE ( 'NONE', *, *, #2200, .F. ) ;
#2577=DIRECTION ( 'NONE',  ( 0.000000000000000000, 1.000000000000000000, 0.000000000000000000 ) ) ;
#2589=CARTESIAN_POINT ( 'NONE',  ( 5.062658757011870954E-16, -2.500000000000000444, 4.133974596215571395 ) ) ;
#2592=DIRECTION ( 'NONE',  ( 0.000000000000000000, -1.000000000000000000, 0.000000000000000000 ) ) ;
#2598=AXIS2_PLACEMENT_3D ( 'NONE', #329, #126, #983 ) ;
#2599=( NAMED_UNIT ( * ) PLANE_ANGLE_UNIT ( ) SI_UNIT ( $, .RADIAN. ) );
#2600=DIRECTION ( 'NONE',  ( 0.4999999999999996114, 0.000000000000000000, -0.8660254037844389297 ) ) ;
#2601=VECTOR ( 'NONE', #2435, 1000.000000000000000 ) ;
#2607=CIRCLE ( 'NONE', #894, 4.171999999999999709 ) ;
#2617=DIRECTION ( 'NONE',  ( 0.000000000000000000, 0.000000000000000000, 1.000000000000000000 ) ) ;
#2620=AXIS2_PLACEMENT_3D ( 'NONE', #1078, #1094, #2039 ) ;
#2622=PRODUCT_DEFINITION_CONTEXT ( 'detailed design', #2424, 'design' ) ;
#2630=DIRECTION ( 'NONE',  ( 0.000000000000000000, 0.000000000000000000, -1.000000000000000000 ) ) ;
#2631=ORIENTED_EDGE ( 'NONE', *, *, #579, .F. ) ;
#2639=EDGE_CURVE ( 'NONE', #2728, #53, #1398, .T. ) ;
#2643=CARTESIAN_POINT ( 'NONE',  ( 0.000000000000000000, 3.000000000000000000, 0.000000000000000000 ) ) ;
#2644=VERTEX_POINT ( 'NONE', #2080 ) ;
#2646=CARTESIAN_POINT ( 'NONE',  ( 0.000000000000000000, 0.000000000000000000, 0.000000000000000000 ) ) ;
#2651=EDGE_CURVE ( 'NONE', #1371, #1727, #1661, .T. ) ;
#2652=AXIS2_PLACEMENT_3D ( 'NONE', #231, #2031, #1309 ) ;
#2653=VERTEX_POINT ( 'NONE', #992 ) ;
#2658=ORIENTED_EDGE ( 'NONE', *, *, #1840, .F. ) ;
#2661=PLANE ( 'NONE',  #882 ) ;
#2662=EDGE_LOOP ( 'NONE', ( #2521, #2126, #1664, #2464, #1207, #1006 ) ) ;
#2665=LINE ( 'NONE', #1798, #2084 ) ;
#2673=ORIENTED_EDGE ( 'NONE', *, *, #1505, .T. ) ;
#2678=ORIENTED_EDGE ( 'NONE', *, *, #2247, .T. ) ;
#2684=CARTESIAN_POINT ( 'NONE',  ( -5.773502691896248429, 13.00000000000000178, 10.00000000000000178 ) ) ;
#2691=DIRECTION ( 'NONE',  ( -0.4999999999999998890, 0.000000000000000000, -0.8660254037844385966 ) ) ;
#2693=ORIENTED_EDGE ( 'NONE', *, *, #164, .F. ) ;
#2694=ADVANCED_FACE ( 'NONE', ( #2109 ), #312, .F. ) ;
#2699=ADVANCED_FACE ( 'NONE', ( #1674, #1879 ), #950, .T. ) ;
#2702=AXIS2_PLACEMENT_3D ( 'NONE', #1040, #1944, #1437 ) ;
#2708=DIRECTION ( 'NONE',  ( 0.000000000000000000, -1.000000000000000000, 0.000000000000000000 ) ) ;
#2714=DIRECTION ( 'NONE',  ( -3.004629197474320528E-16, 0.000000000000000000, -1.000000000000000000 ) ) ;
#2715=ORIENTED_EDGE ( 'NONE', *, *, #1412, .T. ) ;
#2721=ADVANCED_FACE ( 'NONE', ( #548 ), #145, .F. ) ;
#2722=EDGE_CURVE ( 'NONE', #2728, #2653, #1362, .T. ) ;
#2725=ORIENTED_EDGE ( 'NONE', *, *, #1914, .T. ) ;
#2726=CARTESIAN_POINT ( 'NONE',  ( 0.000000000000000000, 3.000000000000000000, 0.000000000000000000 ) ) ;
#2727=FILL_AREA_STYLE ('',( #207 ) ) ;
#2728=VERTEX_POINT ( 'NONE', #2559 ) ;
#2729=CARTESIAN_POINT ( 'NONE',  ( -5.773502691896248429, 13.00000000000000178, 10.00000000000000178 ) ) ;
#2731=DIRECTION ( 'NONE',  ( 0.5000000000000004441, 0.000000000000000000, 0.8660254037844383745 ) ) ;
#2732=EDGE_CURVE ( 'NONE', #705, #1503, #1829, .T. ) ;
#2735=ADVANCED_FACE ( 'NONE', ( #2759 ), #710, .F. ) ;
#2743=FACE_OUTER_BOUND ( 'NONE', #1279, .T. ) ;
#2746=DIRECTION ( 'NONE',  ( 0.000000000000000000, -1.000000000000000000, 0.000000000000000000 ) ) ;
#2749=VERTEX_POINT ( 'NONE', #2404 ) ;
#2752=DIRECTION ( 'NONE',  ( 0.000000000000000000, 1.000000000000000000, 0.000000000000000000 ) ) ;
#2754=ORIENTED_EDGE ( 'NONE', *, *, #4, .T. ) ;
#2759=FACE_OUTER_BOUND ( 'NONE', #1060, .T. ) ;
#2760=DIRECTION ( 'NONE',  ( -0.4999999999999998890, 0.000000000000000000, -0.8660254037844385966 ) ) ;
#2764=AXIS2_PLACEMENT_3D ( 'NONE', #2386, #301, #2421 ) ;
#2768=VECTOR ( 'NONE', #18, 1000.000000000000000 ) ;
#2771=ORIENTED_EDGE ( 'NONE', *, *, #2651, .T. ) ;
#2774=DIRECTION ( 'NONE',  ( 0.000000000000000000, 0.000000000000000000, 1.000000000000000000 ) ) ;
#2775=ADVANCED_FACE ( 'NONE', ( #360 ), #1500, .T. ) ;
#2776=CARTESIAN_POINT ( 'NONE',  ( 5.773502691896257311, 3.000000000000000000, -10.00000000000000000 ) ) ;
#2777=ORIENTED_EDGE ( 'NONE', *, *, #1451, .F. ) ;
#2778=CARTESIAN_POINT ( 'NONE',  ( 0.000000000000000000, -2.500000000000000444, 0.000000000000000000 ) ) ;
#2783=EDGE_CURVE ( 'NONE', #81, #2433, #240, .T. ) ;
#2786=EDGE_LOOP ( 'NONE', ( #2902, #2715, #1982, #1457 ) ) ;
#2796=ORIENTED_EDGE ( 'NONE', *, *, #1132, .F. ) ;
#2803=CARTESIAN_POINT ( 'NONE',  ( -11.54700538379251107, 13.00000000000000178, 3.469741003519073858E-15 ) ) ;
#2805=VECTOR ( 'NONE', #1281, 1000.000000000000114 ) ;
#2809=DIRECTION ( 'NONE',  ( 0.000000000000000000, -0.000000000000000000, 1.000000000000000000 ) ) ;
#2810=AXIS2_PLACEMENT_3D ( 'NONE', #2886, #686, #1624 ) ;
#2818=LINE ( 'NONE', #1930, #507 ) ;
#2821=CARTESIAN_POINT ( 'NONE',  ( 6.123233995736766282E-16, 0.000000000000000000, -5.000000000000000000 ) ) ;
#2823=DIRECTION ( 'NONE',  ( 6.123233995737019950E-17, -0.8660254037844267172, 0.5000000000000207612 ) ) ;
#2825=ORIENTED_EDGE ( 'NONE', *, *, #164, .T. ) ;
#2832=DIRECTION ( 'NONE',  ( -0.000000000000000000, 1.000000000000000000, -0.000000000000000000 ) ) ;
#2835=LINE ( 'NONE', #1901, #1118 ) ;
#2837=CARTESIAN_POINT ( 'NONE',  ( -5.773502691896248429, 13.00000000000000178, 10.00000000000000178 ) ) ;
#2839=VERTEX_POINT ( 'NONE', #1045 ) ;
#2843=( GEOMETRIC_REPRESENTATION_CONTEXT ( 3 ) GLOBAL_UNCERTAINTY_ASSIGNED_CONTEXT ( ( #1209 ) ) GLOBAL_UNIT_ASSIGNED_CONTEXT ( ( #1985, #1580, #431 ) ) REPRESENTATION_CONTEXT ( 'NONE', 'WORKASPACE' ) );
#2845=EDGE_CURVE ( 'NONE', #2512, #915, #1950, .T. ) ;
#2849=ORIENTED_EDGE ( 'NONE', *, *, #579, .T. ) ;
#2851=ORIENTED_EDGE ( 'NONE', *, *, #479, .T. ) ;
#2856=VECTOR ( 'NONE', #24, 1000.000000000000000 ) ;
#2857=ORIENTED_EDGE ( 'NONE', *, *, #1560, .F. ) ;
#2859=FACE_OUTER_BOUND ( 'NONE', #1892, .T. ) ;
#2860=DIRECTION ( 'NONE',  ( 0.000000000000000000, 0.000000000000000000, 1.000000000000000000 ) ) ;
#2871=ORIENTED_EDGE ( 'NONE', *, *, #2247, .F. ) ;
#2872=EDGE_CURVE ( 'NONE', #766, #391, #122, .T. ) ;
#2874=CARTESIAN_POINT ( 'NONE',  ( -11.54700538379251107, 3.000000000000000000, 3.469741003519073858E-15 ) ) ;
#2881=ADVANCED_FACE ( 'NONE', ( #2139 ), #1069, .T. ) ;
#2885=AXIS2_PLACEMENT_3D ( 'NONE', #2105, #2752, #1811 ) ;
#2886=CARTESIAN_POINT ( 'NONE',  ( 0.000000000000000000, -3.999999999999900524, 0.000000000000000000 ) ) ;
#2891=AXIS2_PLACEMENT_3D ( 'NONE', #1614, #2393, #2600 ) ;
#2900=DIRECTION ( 'NONE',  ( 0.000000000000000000, 0.000000000000000000, -1.000000000000000000 ) ) ;
#2902=ORIENTED_EDGE ( 'NONE', *, *, #2722, .F. ) ;
#2905=AXIS2_PLACEMENT_3D ( 'NONE', #2298, #1372, #2024 ) ;
#2911=VECTOR ( 'NONE', #2731, 1000.000000000000114 ) ;
#2913=CARTESIAN_POINT ( 'NONE',  ( 0.000000000000000000, 0.000000000000000000, 0.000000000000000000 ) ) ;
#2921=LINE ( 'NONE', #1767, #829 ) ;
#2924=CARTESIAN_POINT ( 'NONE',  ( 6.123233995736766282E-16, -3.999999999999900524, 5.000000000000000000 ) ) ;
#2930=ORIENTED_EDGE ( 'NONE', *, *, #2164, .F. ) ;
#2964=COLOUR_RGB('Black',0.12,0.14,0.17);
#2965=FILL_AREA_STYLE_COLOUR('',#2964);
#2966=FILL_AREA_STYLE('',(#2965));
#2967=SURFACE_STYLE_FILL_AREA(#2966);
#2968=SURFACE_SIDE_STYLE('',(#2967));
#2969=SURFACE_STYLE_USAGE(.BOTH.,#2968);
#2970=PRESENTATION_STYLE_ASSIGNMENT((#2969));
ENDSEC;
END-ISO-10303-21;
